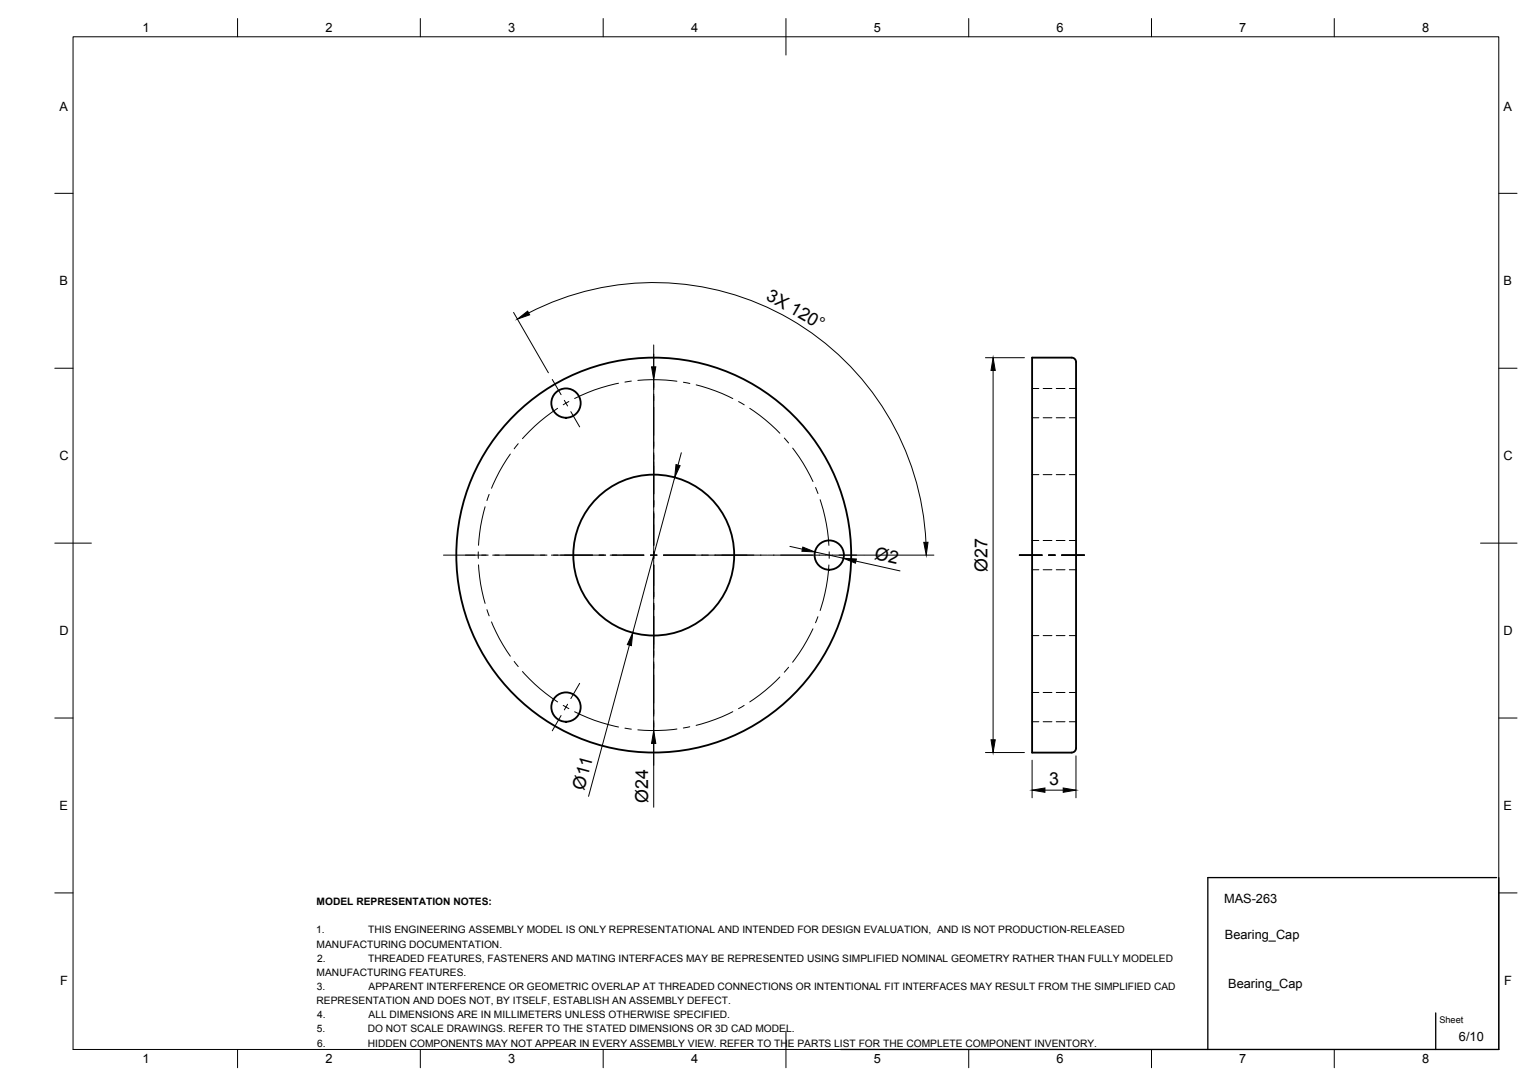
ISO-10303-21;
HEADER;
/* Generated by software containing ST-Developer
 * from STEP Tools, Inc. (www.steptools.com) 
 */

FILE_DESCRIPTION(
/* description */ (''),
/* implementation_level */ '2;1');

FILE_NAME(
/* name */ 'Bearing_Cap.step',
/* time_stamp */ '2026-10-12T15:47:30-07:00',
/* author */ (''),
/* organization */ (''),
/* preprocessor_version */ 'ST-DEVELOPER v20.2',
/* originating_system */ 'Autodesk Translation Framework v15.15.0.0',
/* authorisation */ '');

FILE_SCHEMA (('AUTOMOTIVE_DESIGN { 1 0 10303 214 3 1 1 }'));
ENDSEC;

DATA;
#10=MECHANICAL_DESIGN_GEOMETRIC_PRESENTATION_REPRESENTATION('',(#83),#88483);
#65=SHAPE_REPRESENTATION_RELATIONSHIP('SRR','None',#88521,#74);
#74=ADVANCED_BREP_SHAPE_REPRESENTATION('',(#118),#88475);
#83=STYLED_ITEM('',(#88574),#118);
#118=MANIFOLD_SOLID_BREP('Body1',#12993);
#170=TOROIDAL_SURFACE('',#13723,13.2,0.3);
#349=FACE_BOUND('',#1788,.T.);
#350=FACE_BOUND('',#1789,.T.);
#351=FACE_BOUND('',#1790,.T.);
#352=FACE_BOUND('',#1791,.T.);
#353=FACE_BOUND('',#1794,.T.);
#354=FACE_BOUND('',#1795,.T.);
#355=FACE_BOUND('',#1796,.T.);
#356=FACE_BOUND('',#1797,.T.);
#514=PLANE('',#13730);
#515=PLANE('',#13734);
#1114=FACE_OUTER_BOUND('',#1782,.T.);
#1115=FACE_OUTER_BOUND('',#1783,.T.);
#1116=FACE_OUTER_BOUND('',#1784,.T.);
#1117=FACE_OUTER_BOUND('',#1785,.T.);
#1118=FACE_OUTER_BOUND('',#1786,.T.);
#1119=FACE_OUTER_BOUND('',#1787,.T.);
#1120=FACE_OUTER_BOUND('',#1792,.T.);
#1121=FACE_OUTER_BOUND('',#1793,.T.);
#1782=EDGE_LOOP('',(#10056,#10057,#10058,#10059));
#1783=EDGE_LOOP('',(#10060,#10061,#10062,#10063));
#1784=EDGE_LOOP('',(#10064,#10065,#10066,#10067));
#1785=EDGE_LOOP('',(#10068,#10069,#10070,#10071,#10072));
#1786=EDGE_LOOP('',(#10073,#10074,#10075,#10076,#10077));
#1787=EDGE_LOOP('',(#10078));
#1788=EDGE_LOOP('',(#10079));
#1789=EDGE_LOOP('',(#10080));
#1790=EDGE_LOOP('',(#10081));
#1791=EDGE_LOOP('',(#10082));
#1792=EDGE_LOOP('',(#10083,#10084,#10085,#10086));
#1793=EDGE_LOOP('',(#10087));
#1794=EDGE_LOOP('',(#10088));
#1795=EDGE_LOOP('',(#10089));
#1796=EDGE_LOOP('',(#10090));
#1797=EDGE_LOOP('',(#10091));
#2585=CIRCLE('',#13715,1.);
#2586=CIRCLE('',#13716,1.);
#2587=CIRCLE('',#13718,1.);
#2588=CIRCLE('',#13719,1.);
#2589=CIRCLE('',#13721,1.);
#2590=CIRCLE('',#13722,1.);
#2591=CIRCLE('',#13724,13.2);
#2592=CIRCLE('',#13725,0.3);
#2593=CIRCLE('',#13726,13.5);
#2594=CIRCLE('',#13727,13.5);
#2595=CIRCLE('',#13729,13.5);
#2596=CIRCLE('',#13731,5.5);
#2597=CIRCLE('',#13733,5.5);
#3915=LINE('',#32981,#4385);
#3916=LINE('',#32987,#4386);
#3917=LINE('',#32993,#4387);
#3918=LINE('',#33005,#4388);
#3919=LINE('',#33013,#4389);
#4385=VECTOR('',#15797,1.);
#4386=VECTOR('',#15804,1.);
#4387=VECTOR('',#15811,1.);
#4388=VECTOR('',#15826,13.5);
#4389=VECTOR('',#15837,5.5);
#5291=VERTEX_POINT('',#32978);
#5292=VERTEX_POINT('',#32980);
#5293=VERTEX_POINT('',#32984);
#5294=VERTEX_POINT('',#32986);
#5295=VERTEX_POINT('',#32990);
#5296=VERTEX_POINT('',#32992);
#5297=VERTEX_POINT('',#32996);
#5298=VERTEX_POINT('',#32998);
#5299=VERTEX_POINT('',#33000);
#5300=VERTEX_POINT('',#33004);
#5301=VERTEX_POINT('',#33008);
#5302=VERTEX_POINT('',#33011);
#7040=EDGE_CURVE('',#5291,#5291,#2585,.T.);
#7041=EDGE_CURVE('',#5291,#5292,#3915,.T.);
#7042=EDGE_CURVE('',#5292,#5292,#2586,.T.);
#7043=EDGE_CURVE('',#5293,#5293,#2587,.T.);
#7044=EDGE_CURVE('',#5293,#5294,#3916,.T.);
#7045=EDGE_CURVE('',#5294,#5294,#2588,.T.);
#7046=EDGE_CURVE('',#5295,#5295,#2589,.T.);
#7047=EDGE_CURVE('',#5295,#5296,#3917,.T.);
#7048=EDGE_CURVE('',#5296,#5296,#2590,.T.);
#7049=EDGE_CURVE('',#5297,#5297,#2591,.T.);
#7050=EDGE_CURVE('',#5297,#5298,#2592,.T.);
#7051=EDGE_CURVE('',#5298,#5299,#2593,.T.);
#7052=EDGE_CURVE('',#5299,#5298,#2594,.T.);
#7053=EDGE_CURVE('',#5299,#5300,#3918,.T.);
#7054=EDGE_CURVE('',#5300,#5300,#2595,.T.);
#7055=EDGE_CURVE('',#5301,#5301,#2596,.T.);
#7056=EDGE_CURVE('',#5302,#5302,#2597,.T.);
#7057=EDGE_CURVE('',#5302,#5301,#3919,.T.);
#10056=ORIENTED_EDGE('',*,*,#7040,.F.);
#10057=ORIENTED_EDGE('',*,*,#7041,.T.);
#10058=ORIENTED_EDGE('',*,*,#7042,.F.);
#10059=ORIENTED_EDGE('',*,*,#7041,.F.);
#10060=ORIENTED_EDGE('',*,*,#7043,.F.);
#10061=ORIENTED_EDGE('',*,*,#7044,.T.);
#10062=ORIENTED_EDGE('',*,*,#7045,.F.);
#10063=ORIENTED_EDGE('',*,*,#7044,.F.);
#10064=ORIENTED_EDGE('',*,*,#7046,.F.);
#10065=ORIENTED_EDGE('',*,*,#7047,.T.);
#10066=ORIENTED_EDGE('',*,*,#7048,.F.);
#10067=ORIENTED_EDGE('',*,*,#7047,.F.);
#10068=ORIENTED_EDGE('',*,*,#7049,.T.);
#10069=ORIENTED_EDGE('',*,*,#7050,.T.);
#10070=ORIENTED_EDGE('',*,*,#7051,.T.);
#10071=ORIENTED_EDGE('',*,*,#7052,.T.);
#10072=ORIENTED_EDGE('',*,*,#7050,.F.);
#10073=ORIENTED_EDGE('',*,*,#7052,.F.);
#10074=ORIENTED_EDGE('',*,*,#7053,.T.);
#10075=ORIENTED_EDGE('',*,*,#7054,.T.);
#10076=ORIENTED_EDGE('',*,*,#7053,.F.);
#10077=ORIENTED_EDGE('',*,*,#7051,.F.);
#10078=ORIENTED_EDGE('',*,*,#7049,.F.);
#10079=ORIENTED_EDGE('',*,*,#7040,.T.);
#10080=ORIENTED_EDGE('',*,*,#7043,.T.);
#10081=ORIENTED_EDGE('',*,*,#7046,.T.);
#10082=ORIENTED_EDGE('',*,*,#7055,.T.);
#10083=ORIENTED_EDGE('',*,*,#7056,.T.);
#10084=ORIENTED_EDGE('',*,*,#7057,.T.);
#10085=ORIENTED_EDGE('',*,*,#7055,.F.);
#10086=ORIENTED_EDGE('',*,*,#7057,.F.);
#10087=ORIENTED_EDGE('',*,*,#7054,.F.);
#10088=ORIENTED_EDGE('',*,*,#7042,.T.);
#10089=ORIENTED_EDGE('',*,*,#7045,.T.);
#10090=ORIENTED_EDGE('',*,*,#7048,.T.);
#10091=ORIENTED_EDGE('',*,*,#7056,.F.);
#12164=CYLINDRICAL_SURFACE('',#13714,1.);
#12165=CYLINDRICAL_SURFACE('',#13717,1.);
#12166=CYLINDRICAL_SURFACE('',#13720,1.);
#12167=CYLINDRICAL_SURFACE('',#13728,13.5);
#12168=CYLINDRICAL_SURFACE('',#13732,5.5);
#12644=ADVANCED_FACE('',(#1114),#12164,.F.);
#12645=ADVANCED_FACE('',(#1115),#12165,.F.);
#12646=ADVANCED_FACE('',(#1116),#12166,.F.);
#12647=ADVANCED_FACE('',(#1117),#170,.T.);
#12648=ADVANCED_FACE('',(#1118),#12167,.T.);
#12649=ADVANCED_FACE('',(#1119,#349,#350,#351,#352),#514,.T.);
#12650=ADVANCED_FACE('',(#1120),#12168,.F.);
#12651=ADVANCED_FACE('',(#1121,#353,#354,#355,#356),#515,.F.);
#12993=CLOSED_SHELL('',(#12644,#12645,#12646,#12647,#12648,#12649,#12650,
#12651));
#13713=AXIS2_PLACEMENT_3D('',#32976,#15791,#15792);
#13714=AXIS2_PLACEMENT_3D('',#32977,#15793,#15794);
#13715=AXIS2_PLACEMENT_3D('',#32979,#15795,#15796);
#13716=AXIS2_PLACEMENT_3D('',#32982,#15798,#15799);
#13717=AXIS2_PLACEMENT_3D('',#32983,#15800,#15801);
#13718=AXIS2_PLACEMENT_3D('',#32985,#15802,#15803);
#13719=AXIS2_PLACEMENT_3D('',#32988,#15805,#15806);
#13720=AXIS2_PLACEMENT_3D('',#32989,#15807,#15808);
#13721=AXIS2_PLACEMENT_3D('',#32991,#15809,#15810);
#13722=AXIS2_PLACEMENT_3D('',#32994,#15812,#15813);
#13723=AXIS2_PLACEMENT_3D('',#32995,#15814,#15815);
#13724=AXIS2_PLACEMENT_3D('',#32997,#15816,#15817);
#13725=AXIS2_PLACEMENT_3D('',#32999,#15818,#15819);
#13726=AXIS2_PLACEMENT_3D('',#33001,#15820,#15821);
#13727=AXIS2_PLACEMENT_3D('',#33002,#15822,#15823);
#13728=AXIS2_PLACEMENT_3D('',#33003,#15824,#15825);
#13729=AXIS2_PLACEMENT_3D('',#33006,#15827,#15828);
#13730=AXIS2_PLACEMENT_3D('',#33007,#15829,#15830);
#13731=AXIS2_PLACEMENT_3D('',#33009,#15831,#15832);
#13732=AXIS2_PLACEMENT_3D('',#33010,#15833,#15834);
#13733=AXIS2_PLACEMENT_3D('',#33012,#15835,#15836);
#13734=AXIS2_PLACEMENT_3D('',#33014,#15838,#15839);
#15791=DIRECTION('axis',(0.,0.,1.));
#15792=DIRECTION('refdir',(1.,0.,0.));
#15793=DIRECTION('center_axis',(-1.,0.,0.));
#15794=DIRECTION('ref_axis',(0.,1.,0.));
#15795=DIRECTION('center_axis',(-1.,0.,0.));
#15796=DIRECTION('ref_axis',(0.,1.,0.));
#15797=DIRECTION('',(-1.,0.,0.));
#15798=DIRECTION('center_axis',(1.,0.,0.));
#15799=DIRECTION('ref_axis',(0.,1.,0.));
#15800=DIRECTION('center_axis',(-1.,0.,0.));
#15801=DIRECTION('ref_axis',(0.,1.,0.));
#15802=DIRECTION('center_axis',(-1.,0.,0.));
#15803=DIRECTION('ref_axis',(0.,1.,0.));
#15804=DIRECTION('',(-1.,0.,0.));
#15805=DIRECTION('center_axis',(1.,0.,0.));
#15806=DIRECTION('ref_axis',(0.,1.,0.));
#15807=DIRECTION('center_axis',(-1.,0.,0.));
#15808=DIRECTION('ref_axis',(0.,1.,0.));
#15809=DIRECTION('center_axis',(-1.,0.,0.));
#15810=DIRECTION('ref_axis',(0.,1.,0.));
#15811=DIRECTION('',(-1.,0.,0.));
#15812=DIRECTION('center_axis',(1.,0.,0.));
#15813=DIRECTION('ref_axis',(0.,1.,0.));
#15814=DIRECTION('center_axis',(1.,0.,0.));
#15815=DIRECTION('ref_axis',(0.,0.,-1.));
#15816=DIRECTION('center_axis',(-1.,0.,0.));
#15817=DIRECTION('ref_axis',(0.,0.342020143325669,0.939692620785908));
#15818=DIRECTION('center_axis',(0.,-1.,0.));
#15819=DIRECTION('ref_axis',(0.,0.,1.));
#15820=DIRECTION('center_axis',(1.,0.,0.));
#15821=DIRECTION('ref_axis',(0.,0.342020143325669,0.939692620785908));
#15822=DIRECTION('center_axis',(1.,0.,0.));
#15823=DIRECTION('ref_axis',(0.,0.342020143325669,0.939692620785908));
#15824=DIRECTION('center_axis',(1.,0.,0.));
#15825=DIRECTION('ref_axis',(0.,-0.296296296296299,-0.955096070979823));
#15826=DIRECTION('',(-1.,0.,0.));
#15827=DIRECTION('center_axis',(1.,0.,0.));
#15828=DIRECTION('ref_axis',(0.,-0.296296296296299,-0.955096070979823));
#15829=DIRECTION('center_axis',(1.,0.,0.));
#15830=DIRECTION('ref_axis',(0.,1.,0.));
#15831=DIRECTION('center_axis',(-1.,0.,0.));
#15832=DIRECTION('ref_axis',(0.,1.,0.));
#15833=DIRECTION('center_axis',(1.,0.,0.));
#15834=DIRECTION('ref_axis',(0.,1.,0.));
#15835=DIRECTION('center_axis',(-1.,0.,0.));
#15836=DIRECTION('ref_axis',(0.,1.,0.));
#15837=DIRECTION('',(1.,0.,0.));
#15838=DIRECTION('center_axis',(1.,0.,0.));
#15839=DIRECTION('ref_axis',(0.,1.,0.));
#32976=CARTESIAN_POINT('',(0.,0.,0.));
#32977=CARTESIAN_POINT('Origin',(26.3408711739,15.6090782051017,5.99920149541289));
#32978=CARTESIAN_POINT('',(26.3408711739,14.6090782051017,5.99920149541289));
#32979=CARTESIAN_POINT('Origin',(26.3408711739,15.6090782051017,5.99920149541289));
#32980=CARTESIAN_POINT('',(23.3408711739,14.6090782051017,5.99920149541289));
#32981=CARTESIAN_POINT('',(26.3408711739,14.6090782051017,5.99920149541289));
#32982=CARTESIAN_POINT('Origin',(23.3408711739,15.6090782051017,5.99920149541289));
#32983=CARTESIAN_POINT('Origin',(26.3408711739,36.3909217948983,5.99920149541289));
#32984=CARTESIAN_POINT('',(26.3408711739,35.3909217948983,5.99920149541289));
#32985=CARTESIAN_POINT('Origin',(26.3408711739,36.3909217948983,5.99920149541289));
#32986=CARTESIAN_POINT('',(23.3408711739,35.3909217948983,5.99920149541289));
#32987=CARTESIAN_POINT('',(26.3408711739,35.3909217948983,5.99920149541289));
#32988=CARTESIAN_POINT('Origin',(23.3408711739,36.3909217948983,5.99920149541289));
#32989=CARTESIAN_POINT('Origin',(26.3408711739,26.,-11.9984029908258));
#32990=CARTESIAN_POINT('',(26.3408711739,25.,-11.9984029908258));
#32991=CARTESIAN_POINT('Origin',(26.3408711739,26.,-11.9984029908258));
#32992=CARTESIAN_POINT('',(23.3408711739,25.,-11.9984029908258));
#32993=CARTESIAN_POINT('',(26.3408711739,25.,-11.9984029908258));
#32994=CARTESIAN_POINT('Origin',(23.3408711739,26.,-11.9984029908258));
#32995=CARTESIAN_POINT('Origin',(26.0408711739,26.,7.77156117237612E-15));
#32996=CARTESIAN_POINT('',(26.3408711739,26.,13.2));
#32997=CARTESIAN_POINT('Origin',(26.3408711739,26.,7.77156117237612E-15));
#32998=CARTESIAN_POINT('',(26.0408711739,26.,13.5));
#32999=CARTESIAN_POINT('Origin',(26.0408711739,26.,13.2));
#33000=CARTESIAN_POINT('',(26.0408711739,30.,12.8937969582276));
#33001=CARTESIAN_POINT('Origin',(26.0408711739,26.,7.77156117237612E-15));
#33002=CARTESIAN_POINT('Origin',(26.0408711739,26.,7.77156117237612E-15));
#33003=CARTESIAN_POINT('Origin',(23.3408711739,26.,7.77156117237612E-15));
#33004=CARTESIAN_POINT('',(23.3408711739,30.,12.8937969582276));
#33005=CARTESIAN_POINT('',(23.3408711739,30.,12.8937969582276));
#33006=CARTESIAN_POINT('Origin',(23.3408711739,26.,7.77156117237612E-15));
#33007=CARTESIAN_POINT('Origin',(26.3408711739,26.,1.11022302462516E-14));
#33008=CARTESIAN_POINT('',(26.3408711739,20.5,7.09800543284508E-15));
#33009=CARTESIAN_POINT('Origin',(26.3408711739,26.,7.77156117237612E-15));
#33010=CARTESIAN_POINT('Origin',(23.3408711739,26.,7.77156117237612E-15));
#33011=CARTESIAN_POINT('',(23.3408711739,20.5,7.09800543284508E-15));
#33012=CARTESIAN_POINT('Origin',(23.3408711739,26.,7.77156117237612E-15));
#33013=CARTESIAN_POINT('',(23.3408711739,20.5,7.09800543284507E-15));
#33014=CARTESIAN_POINT('Origin',(23.3408711739,26.,1.11022302462516E-14));
#88464=UNCERTAINTY_MEASURE_WITH_UNIT(LENGTH_MEASURE(0.01),#88484,
'DISTANCE_ACCURACY_VALUE',
'Maximum model space distance between geometric entities at asserted c
onnectivities');
#88472=UNCERTAINTY_MEASURE_WITH_UNIT(LENGTH_MEASURE(0.01),#88484,
'DISTANCE_ACCURACY_VALUE',
'Maximum model space distance between geometric entities at asserted c
onnectivities');
#88475=(
GEOMETRIC_REPRESENTATION_CONTEXT(3)
GLOBAL_UNCERTAINTY_ASSIGNED_CONTEXT((#88464))
GLOBAL_UNIT_ASSIGNED_CONTEXT((#88484,#88486,#88487))
REPRESENTATION_CONTEXT('','3D')
);
#88483=(
GEOMETRIC_REPRESENTATION_CONTEXT(3)
GLOBAL_UNCERTAINTY_ASSIGNED_CONTEXT((#88472))
GLOBAL_UNIT_ASSIGNED_CONTEXT((#88484,#88486,#88487))
REPRESENTATION_CONTEXT('','3D')
);
#88484=(
LENGTH_UNIT()
NAMED_UNIT(*)
SI_UNIT(.MILLI.,.METRE.)
);
#88486=(
NAMED_UNIT(*)
PLANE_ANGLE_UNIT()
SI_UNIT($,.RADIAN.)
);
#88487=(
NAMED_UNIT(*)
SI_UNIT($,.STERADIAN.)
SOLID_ANGLE_UNIT()
);
#88490=SHAPE_DEFINITION_REPRESENTATION(#88500,#88521);
#88500=PRODUCT_DEFINITION_SHAPE('',$,#88532);
#88521=SHAPE_REPRESENTATION('',(#13713),#88475);
#88529=PRODUCT_DEFINITION_CONTEXT('part definition',#88561,'design');
#88532=PRODUCT_DEFINITION('Bearing_Cap','Bearing_Cap',#88542,#88529);
#88542=PRODUCT_DEFINITION_FORMATION('',$,#88565);
#88561=APPLICATION_CONTEXT(
'Core Data for Automotive Mechanical Design Process');
#88562=PRODUCT_CONTEXT('part definition',#88561,'mechanical');
#88565=PRODUCT('Bearing_Cap','Bearing_Cap',$,(#88562));
#88574=PRESENTATION_STYLE_ASSIGNMENT((#88576));
#88576=SURFACE_STYLE_USAGE(.BOTH.,#88578);
#88578=SURFACE_SIDE_STYLE('',(#88580));
#88580=SURFACE_STYLE_FILL_AREA(#88582);
#88582=FILL_AREA_STYLE('Opaque(160,160,160)',(#88584));
#88584=FILL_AREA_STYLE_COLOUR('Opaque(160,160,160)',#88586);
#88586=COLOUR_RGB('Opaque(160,160,160)', 0.66274510, 0.83137255, 0.94901961);
ENDSEC;
END-ISO-10303-21;
